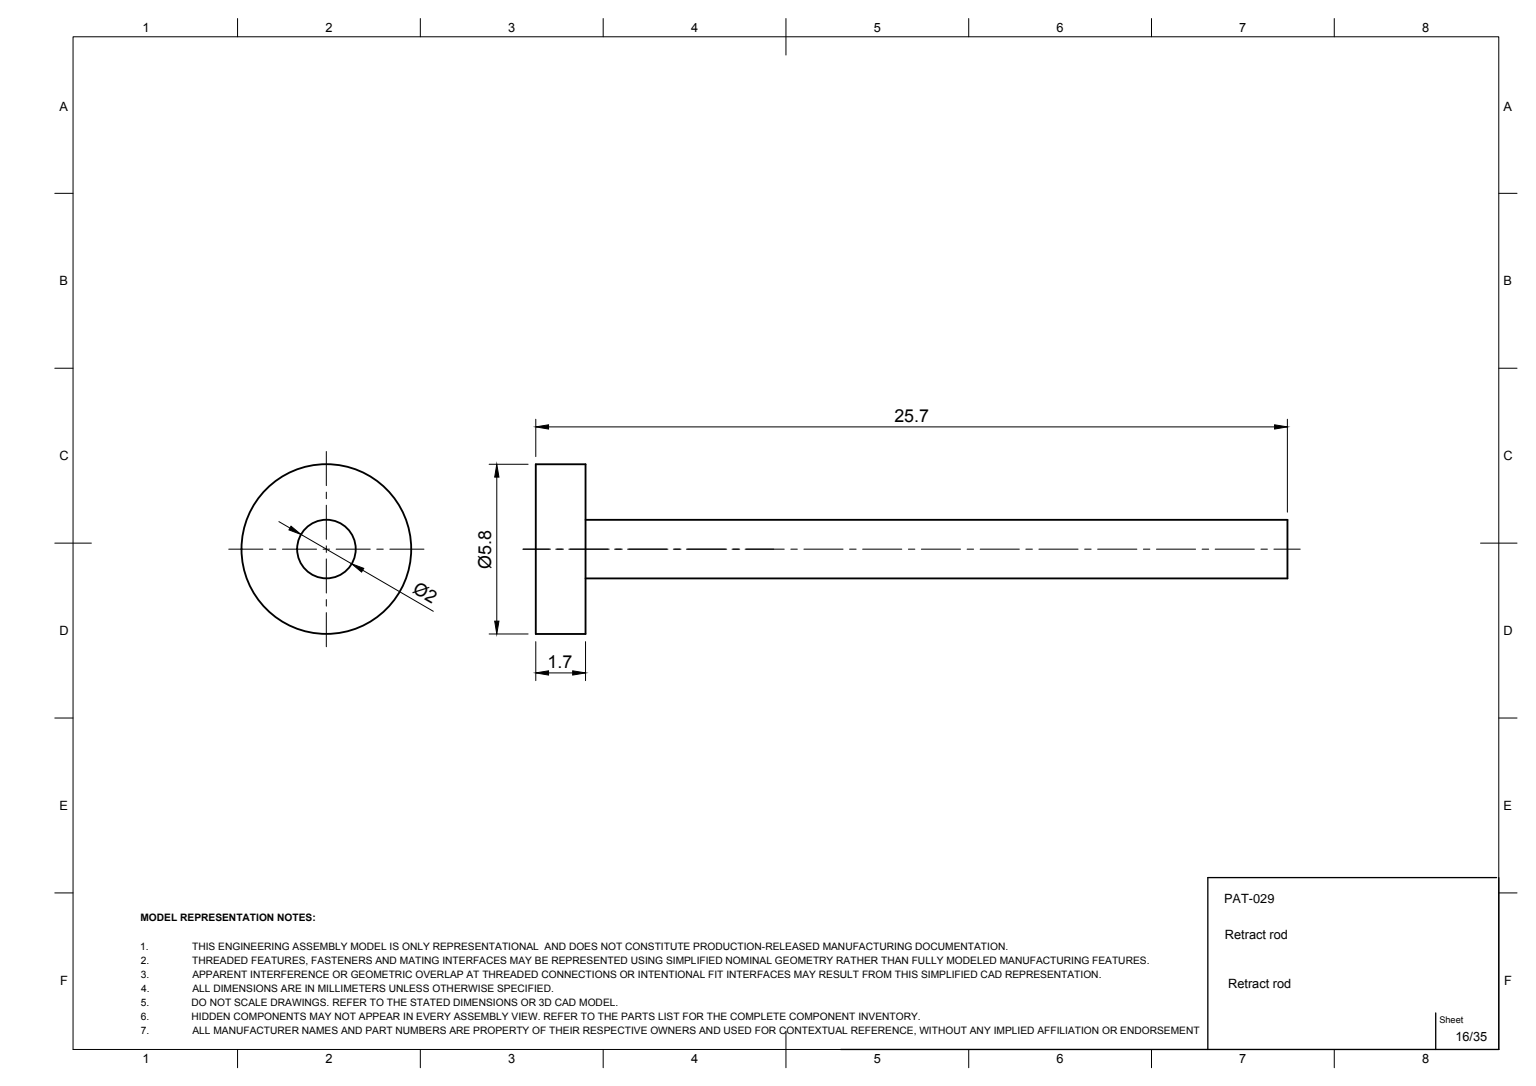
ISO-10303-21;
HEADER;
/* Generated by software containing ST-Developer
 * from STEP Tools, Inc. (www.steptools.com) 
 */

FILE_DESCRIPTION(
/* description */ ('Door-style hinge test fixture with detent'),
/* implementation_level */ '2;1');

FILE_NAME(
/* name */ 'Retract rod.step',
/* time_stamp */ '2026-10-28T03:24:57-07:00',
/* author */ (''),
/* organization */ (''),
/* preprocessor_version */ 'ST-DEVELOPER v20.2',
/* originating_system */ 'Autodesk Translation Framework v15.17.0.0',
/* authorisation */ '');

FILE_SCHEMA (('AUTOMOTIVE_DESIGN { 1 0 10303 214 3 1 1 }'));
ENDSEC;

DATA;
#10=MECHANICAL_DESIGN_GEOMETRIC_PRESENTATION_REPRESENTATION('',(#334),#9813);
#271=SHAPE_REPRESENTATION_RELATIONSHIP('SRR','None',#9948,#302);
#302=ADVANCED_BREP_SHAPE_REPRESENTATION('',(#374),#9791);
#334=STYLED_ITEM('',(#10183),#374);
#374=MANIFOLD_SOLID_BREP('Body1',#4765);
#459=FACE_BOUND('',#1121,.T.);
#570=PLANE('',#5359);
#571=PLANE('',#5366);
#572=PLANE('',#5367);
#775=FACE_OUTER_BOUND('',#1120,.T.);
#776=FACE_OUTER_BOUND('',#1122,.T.);
#777=FACE_OUTER_BOUND('',#1123,.T.);
#778=FACE_OUTER_BOUND('',#1124,.T.);
#779=FACE_OUTER_BOUND('',#1125,.T.);
#1120=EDGE_LOOP('',(#3731));
#1121=EDGE_LOOP('',(#3732));
#1122=EDGE_LOOP('',(#3733,#3734,#3735,#3736));
#1123=EDGE_LOOP('',(#3737,#3738,#3739,#3740));
#1124=EDGE_LOOP('',(#3741));
#1125=EDGE_LOOP('',(#3742));
#1501=LINE('',#7869,#1821);
#1502=LINE('',#7872,#1822);
#1821=VECTOR('',#6370,0.29);
#1822=VECTOR('',#6373,0.1);
#2069=CIRCLE('',#5360,0.29);
#2070=CIRCLE('',#5361,0.1);
#2071=CIRCLE('',#5363,0.29);
#2072=CIRCLE('',#5365,0.1);
#2397=VERTEX_POINT('',#7862);
#2398=VERTEX_POINT('',#7864);
#2399=VERTEX_POINT('',#7867);
#2400=VERTEX_POINT('',#7871);
#2882=EDGE_CURVE('',#2397,#2397,#2069,.T.);
#2883=EDGE_CURVE('',#2398,#2398,#2070,.T.);
#2884=EDGE_CURVE('',#2399,#2399,#2071,.T.);
#2885=EDGE_CURVE('',#2399,#2397,#1501,.T.);
#2886=EDGE_CURVE('',#2398,#2400,#1502,.T.);
#2887=EDGE_CURVE('',#2400,#2400,#2072,.T.);
#3731=ORIENTED_EDGE('',*,*,#2882,.F.);
#3732=ORIENTED_EDGE('',*,*,#2883,.F.);
#3733=ORIENTED_EDGE('',*,*,#2884,.F.);
#3734=ORIENTED_EDGE('',*,*,#2885,.T.);
#3735=ORIENTED_EDGE('',*,*,#2882,.T.);
#3736=ORIENTED_EDGE('',*,*,#2885,.F.);
#3737=ORIENTED_EDGE('',*,*,#2883,.T.);
#3738=ORIENTED_EDGE('',*,*,#2886,.T.);
#3739=ORIENTED_EDGE('',*,*,#2887,.T.);
#3740=ORIENTED_EDGE('',*,*,#2886,.F.);
#3741=ORIENTED_EDGE('',*,*,#2884,.T.);
#3742=ORIENTED_EDGE('',*,*,#2887,.F.);
#4422=CYLINDRICAL_SURFACE('',#5362,0.29);
#4423=CYLINDRICAL_SURFACE('',#5364,0.1);
#4580=ADVANCED_FACE('',(#775,#459),#570,.F.);
#4581=ADVANCED_FACE('',(#776),#4422,.T.);
#4582=ADVANCED_FACE('',(#777),#4423,.T.);
#4583=ADVANCED_FACE('',(#778),#571,.T.);
#4584=ADVANCED_FACE('',(#779),#572,.F.);
#4765=CLOSED_SHELL('',(#4580,#4581,#4582,#4583,#4584));
#5358=AXIS2_PLACEMENT_3D('',#7860,#6358,#6359);
#5359=AXIS2_PLACEMENT_3D('',#7861,#6360,#6361);
#5360=AXIS2_PLACEMENT_3D('',#7863,#6362,#6363);
#5361=AXIS2_PLACEMENT_3D('',#7865,#6364,#6365);
#5362=AXIS2_PLACEMENT_3D('',#7866,#6366,#6367);
#5363=AXIS2_PLACEMENT_3D('',#7868,#6368,#6369);
#5364=AXIS2_PLACEMENT_3D('',#7870,#6371,#6372);
#5365=AXIS2_PLACEMENT_3D('',#7873,#6374,#6375);
#5366=AXIS2_PLACEMENT_3D('',#7874,#6376,#6377);
#5367=AXIS2_PLACEMENT_3D('',#7875,#6378,#6379);
#6358=DIRECTION('axis',(0.,0.,1.));
#6359=DIRECTION('refdir',(1.,0.,0.));
#6360=DIRECTION('center_axis',(0.,1.,0.));
#6361=DIRECTION('ref_axis',(1.,0.,0.));
#6362=DIRECTION('center_axis',(0.,1.,0.));
#6363=DIRECTION('ref_axis',(1.,0.,0.));
#6364=DIRECTION('center_axis',(0.,-1.,0.));
#6365=DIRECTION('ref_axis',(1.,0.,0.));
#6366=DIRECTION('center_axis',(0.,1.,0.));
#6367=DIRECTION('ref_axis',(1.,0.,0.));
#6368=DIRECTION('center_axis',(0.,1.,0.));
#6369=DIRECTION('ref_axis',(1.,0.,0.));
#6370=DIRECTION('',(0.,-1.,0.));
#6371=DIRECTION('center_axis',(0.,1.,0.));
#6372=DIRECTION('ref_axis',(1.,0.,0.));
#6373=DIRECTION('',(0.,-1.,0.));
#6374=DIRECTION('center_axis',(0.,1.,0.));
#6375=DIRECTION('ref_axis',(1.,0.,0.));
#6376=DIRECTION('center_axis',(0.,1.,0.));
#6377=DIRECTION('ref_axis',(1.,0.,0.));
#6378=DIRECTION('center_axis',(0.,1.,0.));
#6379=DIRECTION('ref_axis',(1.,0.,0.));
#7860=CARTESIAN_POINT('',(0.,0.,0.));
#7861=CARTESIAN_POINT('Origin',(0.,-2.6,7.2));
#7862=CARTESIAN_POINT('',(-0.29,-2.6,7.2));
#7863=CARTESIAN_POINT('Origin',(0.,-2.6,7.2));
#7864=CARTESIAN_POINT('',(-0.1,-2.6,7.2));
#7865=CARTESIAN_POINT('Origin',(0.,-2.6,7.2));
#7866=CARTESIAN_POINT('Origin',(0.,-2.6,7.2));
#7867=CARTESIAN_POINT('',(-0.29,-2.43,7.2));
#7868=CARTESIAN_POINT('Origin',(0.,-2.43,7.2));
#7869=CARTESIAN_POINT('',(-0.29,-2.6,7.2));
#7870=CARTESIAN_POINT('Origin',(0.,-5.,7.2));
#7871=CARTESIAN_POINT('',(-0.1,-5.,7.2));
#7872=CARTESIAN_POINT('',(-0.1,-5.,7.2));
#7873=CARTESIAN_POINT('Origin',(0.,-5.,7.2));
#7874=CARTESIAN_POINT('Origin',(0.,-2.43,7.2));
#7875=CARTESIAN_POINT('Origin',(0.,-5.,7.2));
#9755=UNCERTAINTY_MEASURE_WITH_UNIT(LENGTH_MEASURE(0.001),#9814,
'DISTANCE_ACCURACY_VALUE',
'Maximum model space distance between geometric entities at asserted c
onnectivities');
#9777=UNCERTAINTY_MEASURE_WITH_UNIT(LENGTH_MEASURE(0.001),#9814,
'DISTANCE_ACCURACY_VALUE',
'Maximum model space distance between geometric entities at asserted c
onnectivities');
#9791=(
GEOMETRIC_REPRESENTATION_CONTEXT(3)
GLOBAL_UNCERTAINTY_ASSIGNED_CONTEXT((#9755))
GLOBAL_UNIT_ASSIGNED_CONTEXT((#9814,#9816,#9817))
REPRESENTATION_CONTEXT('','3D')
);
#9813=(
GEOMETRIC_REPRESENTATION_CONTEXT(3)
GLOBAL_UNCERTAINTY_ASSIGNED_CONTEXT((#9777))
GLOBAL_UNIT_ASSIGNED_CONTEXT((#9814,#9816,#9817))
REPRESENTATION_CONTEXT('','3D')
);
#9814=(
LENGTH_UNIT()
NAMED_UNIT(*)
SI_UNIT(.CENTI.,.METRE.)
);
#9816=(
NAMED_UNIT(*)
PLANE_ANGLE_UNIT()
SI_UNIT($,.RADIAN.)
);
#9817=(
NAMED_UNIT(*)
SI_UNIT($,.STERADIAN.)
SOLID_ANGLE_UNIT()
);
#9831=SHAPE_DEFINITION_REPRESENTATION(#9866,#9948);
#9866=PRODUCT_DEFINITION_SHAPE('',$,#9984);
#9948=SHAPE_REPRESENTATION('',(#5358),#9791);
#9970=PRODUCT_DEFINITION_CONTEXT('part definition',#10077,'design');
#9984=PRODUCT_DEFINITION('Retract rod','Retract rod',#10019,#9970);
#10019=PRODUCT_DEFINITION_FORMATION('',$,#10092);
#10077=APPLICATION_CONTEXT(
'Core Data for Automotive Mechanical Design Process');
#10078=PRODUCT_CONTEXT('part definition',#10077,'mechanical');
#10092=PRODUCT('Retract rod','Retract rod','Retract rod',(#10078));
#10177=COLOUR_RGB('Grey',0.48,0.52,0.57);
#10178=FILL_AREA_STYLE_COLOUR('',#10177);
#10179=FILL_AREA_STYLE('',(#10178));
#10180=SURFACE_STYLE_FILL_AREA(#10179);
#10181=SURFACE_SIDE_STYLE('',(#10180));
#10182=SURFACE_STYLE_USAGE(.BOTH.,#10181);
#10183=PRESENTATION_STYLE_ASSIGNMENT((#10182));
ENDSEC;
END-ISO-10303-21;
